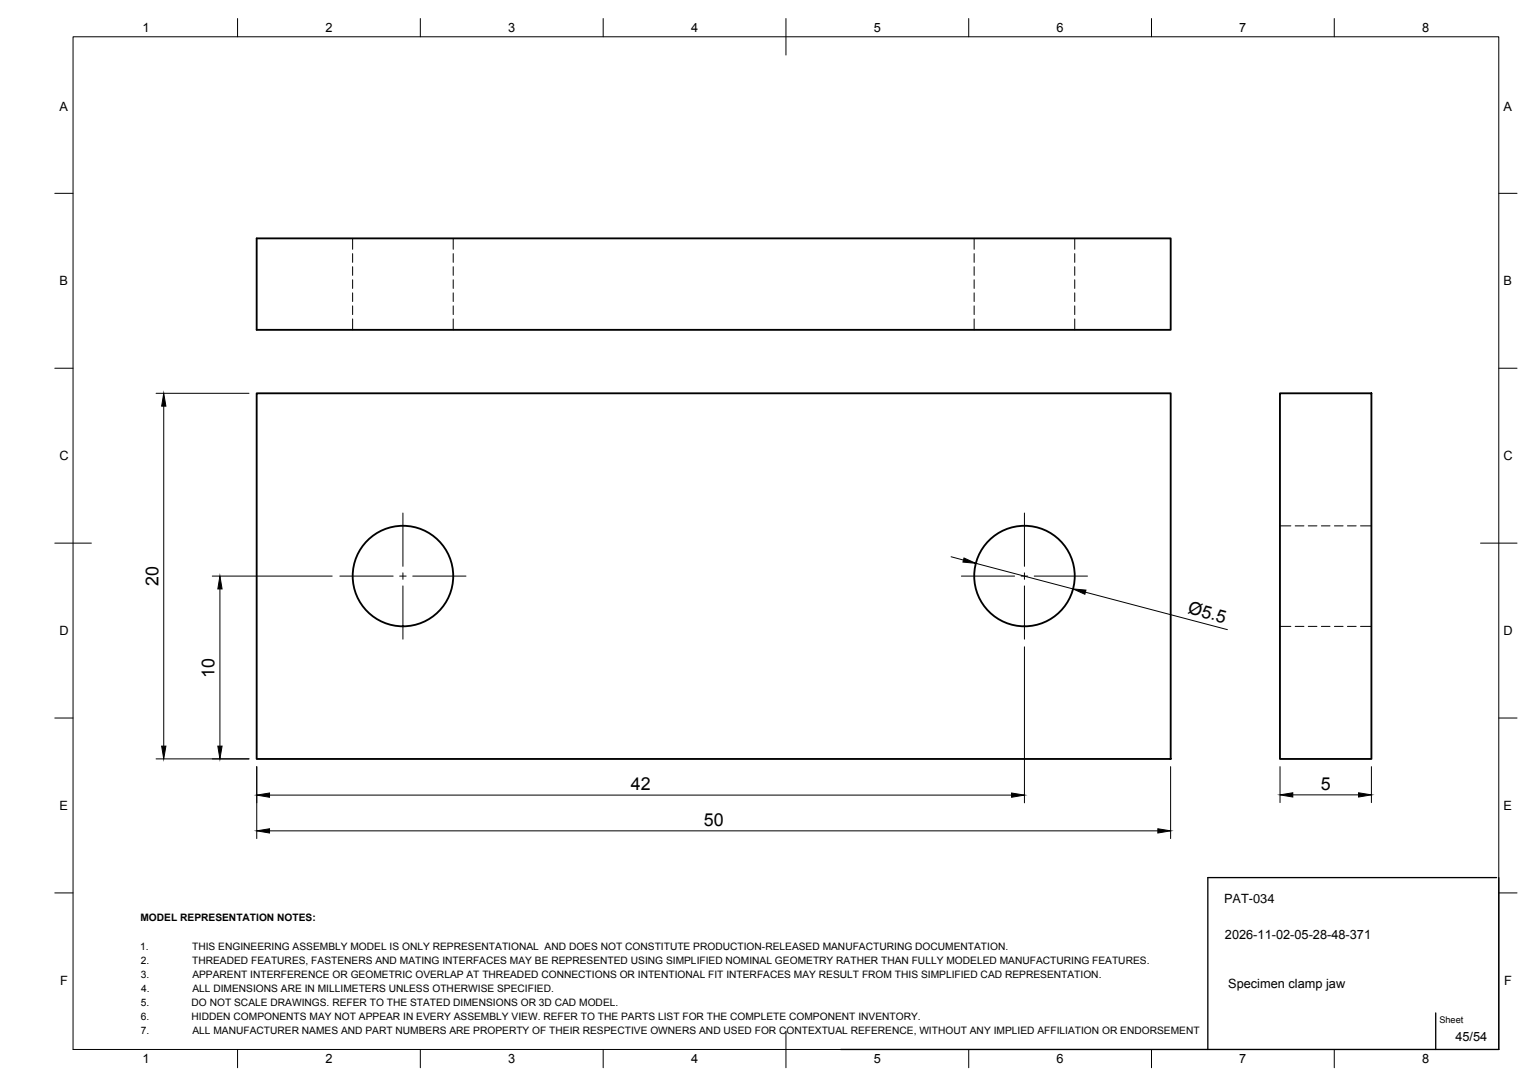
ISO-10303-21;
HEADER;
/* Generated by software containing ST-Developer
 * from STEP Tools, Inc. (www.steptools.com) 
 */

FILE_DESCRIPTION(
/* description */ ('Fatigue rig crank-slider'),
/* implementation_level */ '2;1');

FILE_NAME(
/* name */ 'Specimen clamp jaw.step',
/* time_stamp */ '2026-10-28T03:24:50-07:00',
/* author */ (''),
/* organization */ (''),
/* preprocessor_version */ 'ST-DEVELOPER v20.2',
/* originating_system */ 'Autodesk Translation Framework v15.17.0.0',
/* authorisation */ '');

FILE_SCHEMA (('AUTOMOTIVE_DESIGN { 1 0 10303 214 3 1 1 }'));
ENDSEC;

DATA;
#10=MECHANICAL_DESIGN_GEOMETRIC_PRESENTATION_REPRESENTATION('',(#634),#16911);
#525=SHAPE_REPRESENTATION_RELATIONSHIP('SRR','None',#17169,#575);
#575=ADVANCED_BREP_SHAPE_REPRESENTATION('',(#691),#16898);
#634=STYLED_ITEM('',(#17480),#691);
#691=MANIFOLD_SOLID_BREP('Body1',#8927);
#876=FACE_BOUND('',#2323,.T.);
#877=FACE_BOUND('',#2324,.T.);
#878=FACE_BOUND('',#2326,.T.);
#879=FACE_BOUND('',#2327,.T.);
#1128=PLANE('',#10294);
#1129=PLANE('',#10295);
#1130=PLANE('',#10296);
#1131=PLANE('',#10297);
#1132=PLANE('',#10298);
#1133=PLANE('',#10299);
#1617=FACE_OUTER_BOUND('',#2316,.T.);
#1618=FACE_OUTER_BOUND('',#2317,.T.);
#1619=FACE_OUTER_BOUND('',#2318,.T.);
#1620=FACE_OUTER_BOUND('',#2319,.T.);
#1621=FACE_OUTER_BOUND('',#2320,.T.);
#1622=FACE_OUTER_BOUND('',#2321,.T.);
#1623=FACE_OUTER_BOUND('',#2322,.T.);
#1624=FACE_OUTER_BOUND('',#2325,.T.);
#2316=EDGE_LOOP('',(#7666,#7667,#7668,#7669));
#2317=EDGE_LOOP('',(#7670,#7671,#7672,#7673));
#2318=EDGE_LOOP('',(#7674,#7675,#7676,#7677));
#2319=EDGE_LOOP('',(#7678,#7679,#7680,#7681));
#2320=EDGE_LOOP('',(#7682,#7683,#7684,#7685));
#2321=EDGE_LOOP('',(#7686,#7687,#7688,#7689));
#2322=EDGE_LOOP('',(#7690,#7691,#7692,#7693));
#2323=EDGE_LOOP('',(#7694));
#2324=EDGE_LOOP('',(#7695));
#2325=EDGE_LOOP('',(#7696,#7697,#7698,#7699));
#2326=EDGE_LOOP('',(#7700));
#2327=EDGE_LOOP('',(#7701));
#2906=LINE('',#16147,#3552);
#2907=LINE('',#16153,#3553);
#2908=LINE('',#16158,#3554);
#2909=LINE('',#16160,#3555);
#2910=LINE('',#16162,#3556);
#2911=LINE('',#16163,#3557);
#2912=LINE('',#16166,#3558);
#2913=LINE('',#16168,#3559);
#2914=LINE('',#16169,#3560);
#2915=LINE('',#16172,#3561);
#2916=LINE('',#16174,#3562);
#2917=LINE('',#16175,#3563);
#2918=LINE('',#16177,#3564);
#2919=LINE('',#16178,#3565);
#3552=VECTOR('',#12606,0.275);
#3553=VECTOR('',#12613,0.275);
#3554=VECTOR('',#12618,1.);
#3555=VECTOR('',#12619,1.);
#3556=VECTOR('',#12620,1.);
#3557=VECTOR('',#12621,1.);
#3558=VECTOR('',#12624,1.);
#3559=VECTOR('',#12625,1.);
#3560=VECTOR('',#12626,1.);
#3561=VECTOR('',#12629,1.);
#3562=VECTOR('',#12630,1.);
#3563=VECTOR('',#12631,1.);
#3564=VECTOR('',#12634,1.);
#3565=VECTOR('',#12635,1.);
#4087=CIRCLE('',#10289,0.275);
#4088=CIRCLE('',#10290,0.275);
#4089=CIRCLE('',#10292,0.275);
#4090=CIRCLE('',#10293,0.275);
#4723=VERTEX_POINT('',#16144);
#4724=VERTEX_POINT('',#16146);
#4725=VERTEX_POINT('',#16150);
#4726=VERTEX_POINT('',#16152);
#4727=VERTEX_POINT('',#16156);
#4728=VERTEX_POINT('',#16157);
#4729=VERTEX_POINT('',#16159);
#4730=VERTEX_POINT('',#16161);
#4731=VERTEX_POINT('',#16165);
#4732=VERTEX_POINT('',#16167);
#4733=VERTEX_POINT('',#16171);
#4734=VERTEX_POINT('',#16173);
#5731=EDGE_CURVE('',#4723,#4723,#4087,.T.);
#5732=EDGE_CURVE('',#4723,#4724,#2906,.T.);
#5733=EDGE_CURVE('',#4724,#4724,#4088,.T.);
#5734=EDGE_CURVE('',#4725,#4725,#4089,.T.);
#5735=EDGE_CURVE('',#4725,#4726,#2907,.T.);
#5736=EDGE_CURVE('',#4726,#4726,#4090,.T.);
#5737=EDGE_CURVE('',#4727,#4728,#2908,.T.);
#5738=EDGE_CURVE('',#4728,#4729,#2909,.T.);
#5739=EDGE_CURVE('',#4730,#4729,#2910,.T.);
#5740=EDGE_CURVE('',#4727,#4730,#2911,.T.);
#5741=EDGE_CURVE('',#4731,#4727,#2912,.T.);
#5742=EDGE_CURVE('',#4732,#4730,#2913,.T.);
#5743=EDGE_CURVE('',#4731,#4732,#2914,.T.);
#5744=EDGE_CURVE('',#4733,#4731,#2915,.T.);
#5745=EDGE_CURVE('',#4734,#4732,#2916,.T.);
#5746=EDGE_CURVE('',#4733,#4734,#2917,.T.);
#5747=EDGE_CURVE('',#4728,#4733,#2918,.T.);
#5748=EDGE_CURVE('',#4729,#4734,#2919,.T.);
#7666=ORIENTED_EDGE('',*,*,#5731,.F.);
#7667=ORIENTED_EDGE('',*,*,#5732,.T.);
#7668=ORIENTED_EDGE('',*,*,#5733,.F.);
#7669=ORIENTED_EDGE('',*,*,#5732,.F.);
#7670=ORIENTED_EDGE('',*,*,#5734,.F.);
#7671=ORIENTED_EDGE('',*,*,#5735,.T.);
#7672=ORIENTED_EDGE('',*,*,#5736,.F.);
#7673=ORIENTED_EDGE('',*,*,#5735,.F.);
#7674=ORIENTED_EDGE('',*,*,#5737,.T.);
#7675=ORIENTED_EDGE('',*,*,#5738,.T.);
#7676=ORIENTED_EDGE('',*,*,#5739,.F.);
#7677=ORIENTED_EDGE('',*,*,#5740,.F.);
#7678=ORIENTED_EDGE('',*,*,#5741,.T.);
#7679=ORIENTED_EDGE('',*,*,#5740,.T.);
#7680=ORIENTED_EDGE('',*,*,#5742,.F.);
#7681=ORIENTED_EDGE('',*,*,#5743,.F.);
#7682=ORIENTED_EDGE('',*,*,#5744,.T.);
#7683=ORIENTED_EDGE('',*,*,#5743,.T.);
#7684=ORIENTED_EDGE('',*,*,#5745,.F.);
#7685=ORIENTED_EDGE('',*,*,#5746,.F.);
#7686=ORIENTED_EDGE('',*,*,#5747,.T.);
#7687=ORIENTED_EDGE('',*,*,#5746,.T.);
#7688=ORIENTED_EDGE('',*,*,#5748,.F.);
#7689=ORIENTED_EDGE('',*,*,#5738,.F.);
#7690=ORIENTED_EDGE('',*,*,#5748,.T.);
#7691=ORIENTED_EDGE('',*,*,#5745,.T.);
#7692=ORIENTED_EDGE('',*,*,#5742,.T.);
#7693=ORIENTED_EDGE('',*,*,#5739,.T.);
#7694=ORIENTED_EDGE('',*,*,#5733,.T.);
#7695=ORIENTED_EDGE('',*,*,#5736,.T.);
#7696=ORIENTED_EDGE('',*,*,#5747,.F.);
#7697=ORIENTED_EDGE('',*,*,#5737,.F.);
#7698=ORIENTED_EDGE('',*,*,#5741,.F.);
#7699=ORIENTED_EDGE('',*,*,#5744,.F.);
#7700=ORIENTED_EDGE('',*,*,#5731,.T.);
#7701=ORIENTED_EDGE('',*,*,#5734,.T.);
#8332=CYLINDRICAL_SURFACE('',#10288,0.275);
#8333=CYLINDRICAL_SURFACE('',#10291,0.275);
#8755=ADVANCED_FACE('',(#1617),#8332,.F.);
#8756=ADVANCED_FACE('',(#1618),#8333,.F.);
#8757=ADVANCED_FACE('',(#1619),#1128,.T.);
#8758=ADVANCED_FACE('',(#1620),#1129,.T.);
#8759=ADVANCED_FACE('',(#1621),#1130,.T.);
#8760=ADVANCED_FACE('',(#1622),#1131,.T.);
#8761=ADVANCED_FACE('',(#1623,#876,#877),#1132,.T.);
#8762=ADVANCED_FACE('',(#1624,#878,#879),#1133,.F.);
#8927=CLOSED_SHELL('',(#8755,#8756,#8757,#8758,#8759,#8760,#8761,#8762));
#10287=AXIS2_PLACEMENT_3D('',#16142,#12600,#12601);
#10288=AXIS2_PLACEMENT_3D('',#16143,#12602,#12603);
#10289=AXIS2_PLACEMENT_3D('',#16145,#12604,#12605);
#10290=AXIS2_PLACEMENT_3D('',#16148,#12607,#12608);
#10291=AXIS2_PLACEMENT_3D('',#16149,#12609,#12610);
#10292=AXIS2_PLACEMENT_3D('',#16151,#12611,#12612);
#10293=AXIS2_PLACEMENT_3D('',#16154,#12614,#12615);
#10294=AXIS2_PLACEMENT_3D('',#16155,#12616,#12617);
#10295=AXIS2_PLACEMENT_3D('',#16164,#12622,#12623);
#10296=AXIS2_PLACEMENT_3D('',#16170,#12627,#12628);
#10297=AXIS2_PLACEMENT_3D('',#16176,#12632,#12633);
#10298=AXIS2_PLACEMENT_3D('',#16179,#12636,#12637);
#10299=AXIS2_PLACEMENT_3D('',#16180,#12638,#12639);
#12600=DIRECTION('axis',(0.,0.,1.));
#12601=DIRECTION('refdir',(1.,0.,0.));
#12602=DIRECTION('center_axis',(0.,0.,1.));
#12603=DIRECTION('ref_axis',(1.,0.,0.));
#12604=DIRECTION('center_axis',(0.,0.,1.));
#12605=DIRECTION('ref_axis',(1.,0.,0.));
#12606=DIRECTION('',(0.,0.,1.));
#12607=DIRECTION('center_axis',(0.,0.,-1.));
#12608=DIRECTION('ref_axis',(1.,0.,0.));
#12609=DIRECTION('center_axis',(0.,0.,1.));
#12610=DIRECTION('ref_axis',(1.,0.,0.));
#12611=DIRECTION('center_axis',(0.,0.,1.));
#12612=DIRECTION('ref_axis',(1.,0.,0.));
#12613=DIRECTION('',(0.,0.,1.));
#12614=DIRECTION('center_axis',(0.,0.,-1.));
#12615=DIRECTION('ref_axis',(1.,0.,0.));
#12616=DIRECTION('center_axis',(0.,1.,0.));
#12617=DIRECTION('ref_axis',(-1.,0.,0.));
#12618=DIRECTION('',(-1.,0.,0.));
#12619=DIRECTION('',(0.,0.,1.));
#12620=DIRECTION('',(-1.,0.,0.));
#12621=DIRECTION('',(0.,0.,1.));
#12622=DIRECTION('center_axis',(1.,0.,0.));
#12623=DIRECTION('ref_axis',(0.,1.,0.));
#12624=DIRECTION('',(0.,1.,0.));
#12625=DIRECTION('',(0.,1.,0.));
#12626=DIRECTION('',(0.,0.,1.));
#12627=DIRECTION('center_axis',(0.,-1.,0.));
#12628=DIRECTION('ref_axis',(1.,0.,0.));
#12629=DIRECTION('',(1.,0.,0.));
#12630=DIRECTION('',(1.,0.,0.));
#12631=DIRECTION('',(0.,0.,1.));
#12632=DIRECTION('center_axis',(-1.,0.,0.));
#12633=DIRECTION('ref_axis',(0.,-1.,0.));
#12634=DIRECTION('',(0.,-1.,0.));
#12635=DIRECTION('',(0.,-1.,0.));
#12636=DIRECTION('center_axis',(0.,0.,1.));
#12637=DIRECTION('ref_axis',(1.,0.,0.));
#12638=DIRECTION('center_axis',(0.,0.,1.));
#12639=DIRECTION('ref_axis',(1.,0.,0.));
#16142=CARTESIAN_POINT('',(0.,0.,0.));
#16143=CARTESIAN_POINT('Origin',(11.,-3.2,8.9));
#16144=CARTESIAN_POINT('',(10.725,-3.2,9.));
#16145=CARTESIAN_POINT('Origin',(11.,-3.2,9.));
#16146=CARTESIAN_POINT('',(10.725,-3.2,9.5));
#16147=CARTESIAN_POINT('',(10.725,-3.2,8.9));
#16148=CARTESIAN_POINT('Origin',(11.,-3.2,9.5));
#16149=CARTESIAN_POINT('Origin',(11.,0.2,8.9));
#16150=CARTESIAN_POINT('',(10.725,0.2,9.));
#16151=CARTESIAN_POINT('Origin',(11.,0.2,9.));
#16152=CARTESIAN_POINT('',(10.725,0.2,9.5));
#16153=CARTESIAN_POINT('',(10.725,0.2,8.9));
#16154=CARTESIAN_POINT('Origin',(11.,0.2,9.5));
#16155=CARTESIAN_POINT('Origin',(12.,1.,9.));
#16156=CARTESIAN_POINT('',(12.,1.,9.));
#16157=CARTESIAN_POINT('',(10.,1.,9.));
#16158=CARTESIAN_POINT('',(12.,1.,9.));
#16159=CARTESIAN_POINT('',(10.,1.,9.5));
#16160=CARTESIAN_POINT('',(10.,1.,9.));
#16161=CARTESIAN_POINT('',(12.,1.,9.5));
#16162=CARTESIAN_POINT('',(12.,1.,9.5));
#16163=CARTESIAN_POINT('',(12.,1.,9.));
#16164=CARTESIAN_POINT('Origin',(12.,-4.,9.));
#16165=CARTESIAN_POINT('',(12.,-4.,9.));
#16166=CARTESIAN_POINT('',(12.,-4.,9.));
#16167=CARTESIAN_POINT('',(12.,-4.,9.5));
#16168=CARTESIAN_POINT('',(12.,-4.,9.5));
#16169=CARTESIAN_POINT('',(12.,-4.,9.));
#16170=CARTESIAN_POINT('Origin',(10.,-4.,9.));
#16171=CARTESIAN_POINT('',(10.,-4.,9.));
#16172=CARTESIAN_POINT('',(10.,-4.,9.));
#16173=CARTESIAN_POINT('',(10.,-4.,9.5));
#16174=CARTESIAN_POINT('',(10.,-4.,9.5));
#16175=CARTESIAN_POINT('',(10.,-4.,9.));
#16176=CARTESIAN_POINT('Origin',(10.,1.,9.));
#16177=CARTESIAN_POINT('',(10.,1.,9.));
#16178=CARTESIAN_POINT('',(10.,1.,9.5));
#16179=CARTESIAN_POINT('Origin',(11.,-1.5,9.5));
#16180=CARTESIAN_POINT('Origin',(11.,-1.5,9.));
#16839=UNCERTAINTY_MEASURE_WITH_UNIT(LENGTH_MEASURE(0.001),#16912,
'DISTANCE_ACCURACY_VALUE',
'Maximum model space distance between geometric entities at asserted c
onnectivities');
#16852=UNCERTAINTY_MEASURE_WITH_UNIT(LENGTH_MEASURE(0.001),#16912,
'DISTANCE_ACCURACY_VALUE',
'Maximum model space distance between geometric entities at asserted c
onnectivities');
#16898=(
GEOMETRIC_REPRESENTATION_CONTEXT(3)
GLOBAL_UNCERTAINTY_ASSIGNED_CONTEXT((#16839))
GLOBAL_UNIT_ASSIGNED_CONTEXT((#16912,#16914,#16915))
REPRESENTATION_CONTEXT('','3D')
);
#16911=(
GEOMETRIC_REPRESENTATION_CONTEXT(3)
GLOBAL_UNCERTAINTY_ASSIGNED_CONTEXT((#16852))
GLOBAL_UNIT_ASSIGNED_CONTEXT((#16912,#16914,#16915))
REPRESENTATION_CONTEXT('','3D')
);
#16912=(
LENGTH_UNIT()
NAMED_UNIT(*)
SI_UNIT(.CENTI.,.METRE.)
);
#16914=(
NAMED_UNIT(*)
PLANE_ANGLE_UNIT()
SI_UNIT($,.RADIAN.)
);
#16915=(
NAMED_UNIT(*)
SI_UNIT($,.STERADIAN.)
SOLID_ANGLE_UNIT()
);
#16961=SHAPE_DEFINITION_REPRESENTATION(#17033,#17169);
#17033=PRODUCT_DEFINITION_SHAPE('',$,#17228);
#17169=SHAPE_REPRESENTATION('',(#10287),#16898);
#17182=PRODUCT_DEFINITION_CONTEXT('part definition',#17358,'design');
#17228=PRODUCT_DEFINITION('Specimen clamp jaw','Specimen clamp jaw',#17286,
#17182);
#17286=PRODUCT_DEFINITION_FORMATION('',$,#17405);
#17358=APPLICATION_CONTEXT(
'Core Data for Automotive Mechanical Design Process');
#17359=PRODUCT_CONTEXT('part definition',#17358,'mechanical');
#17405=PRODUCT('Specimen clamp jaw','Specimen clamp jaw',
'Specimen clamp jaw',(#17359));
#17474=COLOUR_RGB('Sky Blue',0.24,0.69,0.87);
#17475=FILL_AREA_STYLE_COLOUR('',#17474);
#17476=FILL_AREA_STYLE('',(#17475));
#17477=SURFACE_STYLE_FILL_AREA(#17476);
#17478=SURFACE_SIDE_STYLE('',(#17477));
#17479=SURFACE_STYLE_USAGE(.BOTH.,#17478);
#17480=PRESENTATION_STYLE_ASSIGNMENT((#17479));
ENDSEC;
END-ISO-10303-21;
